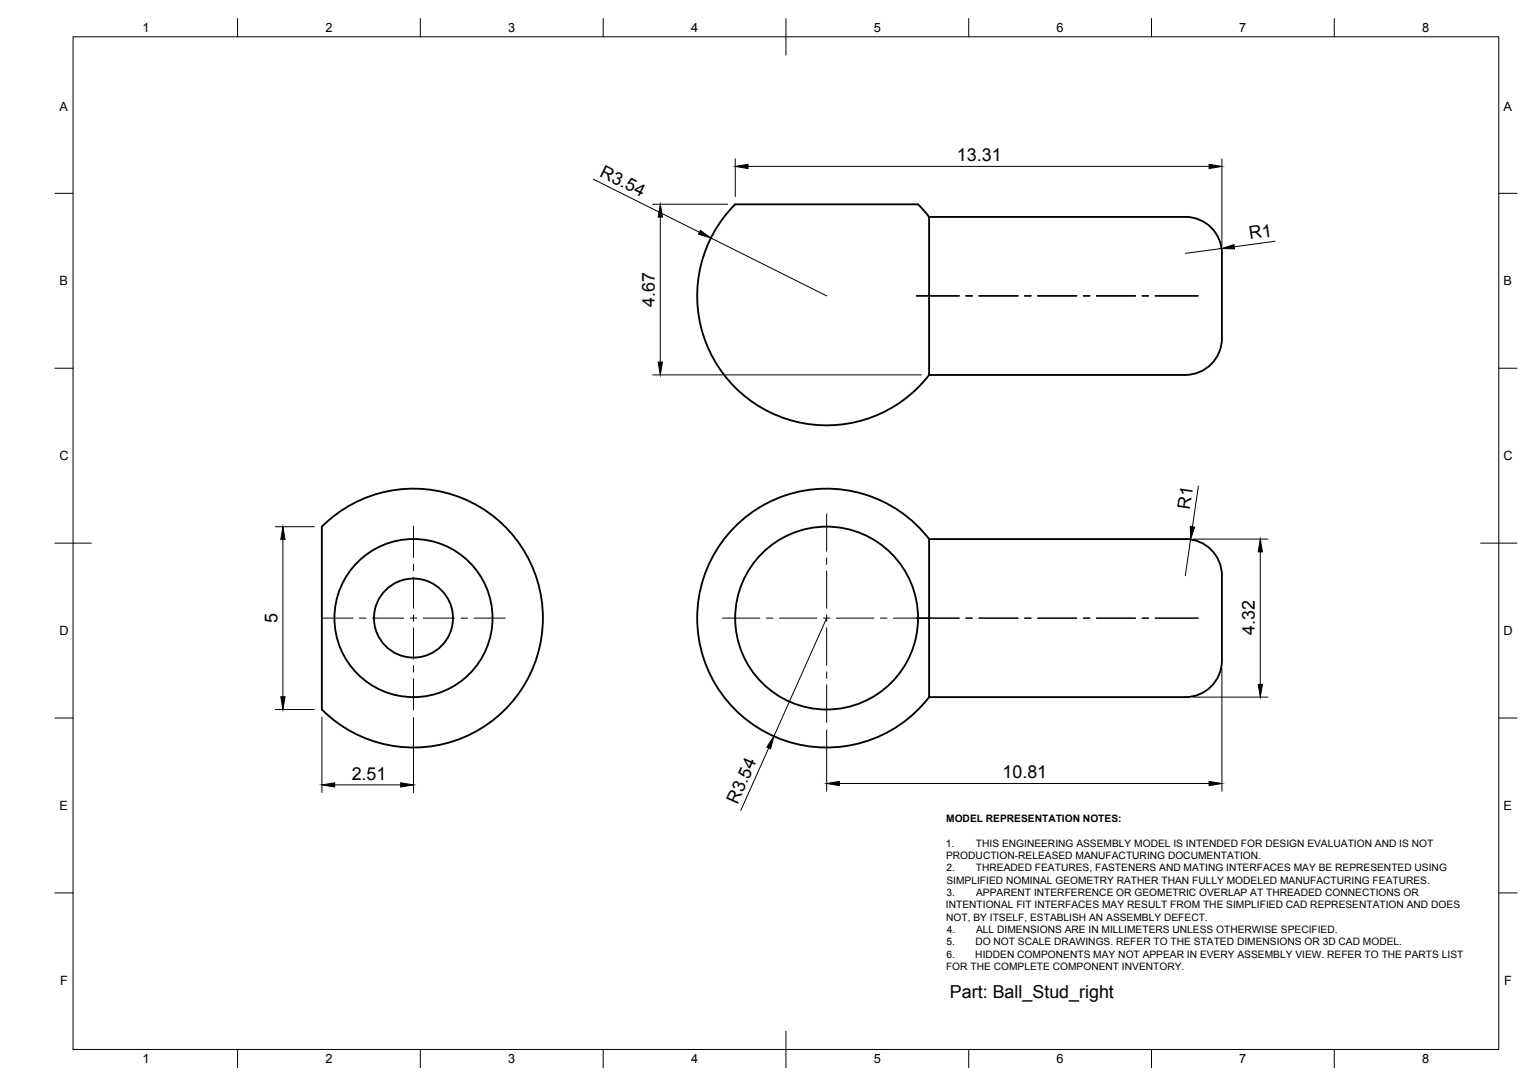
ISO-10303-21;
HEADER;
/* Generated by software containing ST-Developer
 * from STEP Tools, Inc. (www.steptools.com) 
 */

FILE_DESCRIPTION(
/* description */ (''),
/* implementation_level */ '2;1');

FILE_NAME(
/* name */ 'Ball_Stud_right.step',
/* time_stamp */ '2026-10-04T22:13:49-07:00',
/* author */ (''),
/* organization */ (''),
/* preprocessor_version */ 'ST-DEVELOPER v20.2',
/* originating_system */ 'Autodesk Translation Framework v15.15.0.0',
/* authorisation */ '');

FILE_SCHEMA (('AUTOMOTIVE_DESIGN { 1 0 10303 214 3 1 1 }'));
ENDSEC;

DATA;
#10=MECHANICAL_DESIGN_GEOMETRIC_PRESENTATION_REPRESENTATION('',(#364),#40734);
#348=SHAPE_REPRESENTATION_RELATIONSHIP('SRR','None',#40769,#356);
#356=ADVANCED_BREP_SHAPE_REPRESENTATION('',(#373),#40729);
#364=STYLED_ITEM('',(#40815),#373);
#373=MANIFOLD_SOLID_BREP('Body1',#3169);
#380=SPHERICAL_SURFACE('',#3338,3.53951905042299);
#387=FACE_BOUND('',#629,.T.);
#388=FACE_BOUND('',#634,.T.);
#394=TOROIDAL_SURFACE('',#3325,1.16126351211314,1.);
#408=PLANE('',#3324);
#409=PLANE('',#3330);
#410=PLANE('',#3337);
#459=FACE_OUTER_BOUND('',#625,.T.);
#460=FACE_OUTER_BOUND('',#626,.T.);
#461=FACE_OUTER_BOUND('',#627,.T.);
#462=FACE_OUTER_BOUND('',#628,.T.);
#463=FACE_OUTER_BOUND('',#630,.T.);
#464=FACE_OUTER_BOUND('',#631,.T.);
#465=FACE_OUTER_BOUND('',#632,.T.);
#466=FACE_OUTER_BOUND('',#633,.T.);
#625=EDGE_LOOP('',(#2088,#2089,#2090,#2091));
#626=EDGE_LOOP('',(#2092));
#627=EDGE_LOOP('',(#2093,#2094,#2095,#2096,#2097));
#628=EDGE_LOOP('',(#2098));
#629=EDGE_LOOP('',(#2099));
#630=EDGE_LOOP('',(#2100,#2101,#2102,#2103,#2104,#2105));
#631=EDGE_LOOP('',(#2106,#2107,#2108,#2109));
#632=EDGE_LOOP('',(#2110));
#633=EDGE_LOOP('',(#2111,#2112,#2113,#2114));
#634=EDGE_LOOP('',(#2115));
#786=LINE('',#6439,#928);
#787=LINE('',#6453,#929);
#788=LINE('',#6461,#930);
#928=VECTOR('',#3629,1.08063175605657);
#929=VECTOR('',#3648,2.16126351211314);
#930=VECTOR('',#3657,2.5);
#1063=CIRCLE('',#3322,1.08063175605657);
#1064=CIRCLE('',#3323,1.08063175605657);
#1065=CIRCLE('',#3326,1.16126351211314);
#1066=CIRCLE('',#3327,1.);
#1067=CIRCLE('',#3328,2.16126351211314);
#1068=CIRCLE('',#3329,2.16126351211314);
#1069=CIRCLE('',#3332,2.16126351211314);
#1070=CIRCLE('',#3333,2.16126351211314);
#1071=CIRCLE('',#3335,2.5);
#1072=CIRCLE('',#3336,2.5);
#1073=CIRCLE('',#3339,3.53951905042299);
#1149=VERTEX_POINT('',#6436);
#1150=VERTEX_POINT('',#6438);
#1151=VERTEX_POINT('',#6443);
#1152=VERTEX_POINT('',#6445);
#1153=VERTEX_POINT('',#6447);
#1154=VERTEX_POINT('',#6452);
#1155=VERTEX_POINT('',#6454);
#1156=VERTEX_POINT('',#6458);
#1157=VERTEX_POINT('',#6460);
#1158=VERTEX_POINT('',#6465);
#1520=EDGE_CURVE('',#1149,#1149,#1063,.T.);
#1521=EDGE_CURVE('',#1149,#1150,#786,.T.);
#1522=EDGE_CURVE('',#1150,#1150,#1064,.T.);
#1523=EDGE_CURVE('',#1151,#1151,#1065,.T.);
#1524=EDGE_CURVE('',#1151,#1152,#1066,.T.);
#1525=EDGE_CURVE('',#1152,#1153,#1067,.T.);
#1526=EDGE_CURVE('',#1153,#1152,#1068,.T.);
#1527=EDGE_CURVE('',#1153,#1154,#787,.T.);
#1528=EDGE_CURVE('',#1154,#1155,#1069,.T.);
#1529=EDGE_CURVE('',#1155,#1154,#1070,.T.);
#1530=EDGE_CURVE('',#1156,#1156,#1071,.T.);
#1531=EDGE_CURVE('',#1156,#1157,#788,.T.);
#1532=EDGE_CURVE('',#1157,#1157,#1072,.T.);
#1533=EDGE_CURVE('',#1155,#1158,#1073,.T.);
#2088=ORIENTED_EDGE('',*,*,#1520,.F.);
#2089=ORIENTED_EDGE('',*,*,#1521,.T.);
#2090=ORIENTED_EDGE('',*,*,#1522,.T.);
#2091=ORIENTED_EDGE('',*,*,#1521,.F.);
#2092=ORIENTED_EDGE('',*,*,#1522,.F.);
#2093=ORIENTED_EDGE('',*,*,#1523,.T.);
#2094=ORIENTED_EDGE('',*,*,#1524,.T.);
#2095=ORIENTED_EDGE('',*,*,#1525,.T.);
#2096=ORIENTED_EDGE('',*,*,#1526,.T.);
#2097=ORIENTED_EDGE('',*,*,#1524,.F.);
#2098=ORIENTED_EDGE('',*,*,#1523,.F.);
#2099=ORIENTED_EDGE('',*,*,#1520,.T.);
#2100=ORIENTED_EDGE('',*,*,#1526,.F.);
#2101=ORIENTED_EDGE('',*,*,#1527,.T.);
#2102=ORIENTED_EDGE('',*,*,#1528,.T.);
#2103=ORIENTED_EDGE('',*,*,#1529,.T.);
#2104=ORIENTED_EDGE('',*,*,#1527,.F.);
#2105=ORIENTED_EDGE('',*,*,#1525,.F.);
#2106=ORIENTED_EDGE('',*,*,#1530,.T.);
#2107=ORIENTED_EDGE('',*,*,#1531,.T.);
#2108=ORIENTED_EDGE('',*,*,#1532,.F.);
#2109=ORIENTED_EDGE('',*,*,#1531,.F.);
#2110=ORIENTED_EDGE('',*,*,#1530,.F.);
#2111=ORIENTED_EDGE('',*,*,#1529,.F.);
#2112=ORIENTED_EDGE('',*,*,#1533,.T.);
#2113=ORIENTED_EDGE('',*,*,#1533,.F.);
#2114=ORIENTED_EDGE('',*,*,#1528,.F.);
#2115=ORIENTED_EDGE('',*,*,#1532,.T.);
#2905=CYLINDRICAL_SURFACE('',#3321,1.08063175605657);
#2906=CYLINDRICAL_SURFACE('',#3331,2.16126351211314);
#2907=CYLINDRICAL_SURFACE('',#3334,2.5);
#3038=ADVANCED_FACE('',(#459),#2905,.F.);
#3039=ADVANCED_FACE('',(#460),#408,.T.);
#3040=ADVANCED_FACE('',(#461),#394,.T.);
#3041=ADVANCED_FACE('',(#462,#387),#409,.T.);
#3042=ADVANCED_FACE('',(#463),#2906,.T.);
#3043=ADVANCED_FACE('',(#464),#2907,.F.);
#3044=ADVANCED_FACE('',(#465),#410,.F.);
#3045=ADVANCED_FACE('',(#466,#388),#380,.T.);
#3169=CLOSED_SHELL('',(#3038,#3039,#3040,#3041,#3042,#3043,#3044,#3045));
#3320=AXIS2_PLACEMENT_3D('',#6434,#3623,#3624);
#3321=AXIS2_PLACEMENT_3D('',#6435,#3625,#3626);
#3322=AXIS2_PLACEMENT_3D('',#6437,#3627,#3628);
#3323=AXIS2_PLACEMENT_3D('',#6440,#3630,#3631);
#3324=AXIS2_PLACEMENT_3D('',#6441,#3632,#3633);
#3325=AXIS2_PLACEMENT_3D('',#6442,#3634,#3635);
#3326=AXIS2_PLACEMENT_3D('',#6444,#3636,#3637);
#3327=AXIS2_PLACEMENT_3D('',#6446,#3638,#3639);
#3328=AXIS2_PLACEMENT_3D('',#6448,#3640,#3641);
#3329=AXIS2_PLACEMENT_3D('',#6449,#3642,#3643);
#3330=AXIS2_PLACEMENT_3D('',#6450,#3644,#3645);
#3331=AXIS2_PLACEMENT_3D('',#6451,#3646,#3647);
#3332=AXIS2_PLACEMENT_3D('',#6455,#3649,#3650);
#3333=AXIS2_PLACEMENT_3D('',#6456,#3651,#3652);
#3334=AXIS2_PLACEMENT_3D('',#6457,#3653,#3654);
#3335=AXIS2_PLACEMENT_3D('',#6459,#3655,#3656);
#3336=AXIS2_PLACEMENT_3D('',#6462,#3658,#3659);
#3337=AXIS2_PLACEMENT_3D('',#6463,#3660,#3661);
#3338=AXIS2_PLACEMENT_3D('',#6464,#3662,#3663);
#3339=AXIS2_PLACEMENT_3D('',#6466,#3664,#3665);
#3623=DIRECTION('axis',(0.,0.,1.));
#3624=DIRECTION('refdir',(1.,0.,0.));
#3625=DIRECTION('center_axis',(1.,0.,0.));
#3626=DIRECTION('ref_axis',(0.,-1.,0.));
#3627=DIRECTION('center_axis',(1.,0.,1.22464679914735E-16));
#3628=DIRECTION('ref_axis',(0.,-1.,0.));
#3629=DIRECTION('',(1.,0.,0.));
#3630=DIRECTION('center_axis',(1.,0.,0.));
#3631=DIRECTION('ref_axis',(0.,-1.,0.));
#3632=DIRECTION('center_axis',(-1.,0.,0.));
#3633=DIRECTION('ref_axis',(0.,-1.,0.));
#3634=DIRECTION('center_axis',(-1.,0.,-1.22464679914735E-16));
#3635=DIRECTION('ref_axis',(0.,0.,1.));
#3636=DIRECTION('center_axis',(1.,0.,1.22464679914735E-16));
#3637=DIRECTION('ref_axis',(-1.22464679914735E-16,2.13056796687593E-46,
1.));
#3638=DIRECTION('center_axis',(-1.49975978266185E-32,-1.,1.22464679914735E-16));
#3639=DIRECTION('ref_axis',(0.,-1.22464679914735E-16,-1.));
#3640=DIRECTION('center_axis',(-1.,0.,-1.22464679914735E-16));
#3641=DIRECTION('ref_axis',(-1.22464679914735E-16,2.13056796687593E-46,
1.));
#3642=DIRECTION('center_axis',(-1.,0.,-1.22464679914735E-16));
#3643=DIRECTION('ref_axis',(-1.22464679914735E-16,2.13056796687593E-46,
1.));
#3644=DIRECTION('center_axis',(-1.,0.,-1.22464679914735E-16));
#3645=DIRECTION('ref_axis',(1.22464679914735E-16,-1.22464679914735E-16,
-1.));
#3646=DIRECTION('center_axis',(-1.,0.,-1.22464679914735E-16));
#3647=DIRECTION('ref_axis',(1.22464679914735E-16,-1.22464679914735E-16,
-1.));
#3648=DIRECTION('',(1.,0.,1.22464679914735E-16));
#3649=DIRECTION('center_axis',(-1.,0.,-1.22464679914735E-16));
#3650=DIRECTION('ref_axis',(1.22464679914735E-16,-1.22464679914735E-16,
-1.));
#3651=DIRECTION('center_axis',(-1.,0.,-1.22464679914735E-16));
#3652=DIRECTION('ref_axis',(1.22464679914735E-16,-1.22464679914735E-16,
-1.));
#3653=DIRECTION('center_axis',(1.22464679914735E-16,-1.22464679914735E-16,
-1.));
#3654=DIRECTION('ref_axis',(-1.,1.258548236767E-48,-1.22464679914735E-16));
#3655=DIRECTION('center_axis',(-1.22464679914735E-16,1.22464679914735E-16,
1.));
#3656=DIRECTION('ref_axis',(-1.,1.258548236767E-48,-1.22464679914735E-16));
#3657=DIRECTION('',(1.22464679914735E-16,-1.22464679914735E-16,-1.));
#3658=DIRECTION('center_axis',(-1.22464679914735E-16,1.22464679914735E-16,
1.));
#3659=DIRECTION('ref_axis',(-1.,1.258548236767E-48,-1.22464679914735E-16));
#3660=DIRECTION('center_axis',(-1.22464679914735E-16,1.22464679914735E-16,
1.));
#3661=DIRECTION('ref_axis',(-1.,1.258548236767E-48,-1.22464679914735E-16));
#3662=DIRECTION('center_axis',(-1.,1.22464679914735E-16,-1.22464679914735E-16));
#3663=DIRECTION('ref_axis',(0.,1.,-1.22464679914735E-16));
#3664=DIRECTION('center_axis',(-1.22464679914735E-16,2.4492935982947E-16,
1.));
#3665=DIRECTION('ref_axis',(0.,-1.,2.4492935982947E-16));
#6434=CARTESIAN_POINT('',(0.,0.,0.));
#6435=CARTESIAN_POINT('Origin',(85.6487002358236,0.,-8.24265256448471E-15));
#6436=CARTESIAN_POINT('',(85.6487002358236,1.08063175605657,-8.37499178659588E-15));
#6437=CARTESIAN_POINT('Origin',(85.6487002358236,0.,-8.24265256448471E-15));
#6438=CARTESIAN_POINT('',(89.1487002358236,1.08063175605657,-8.37499178659588E-15));
#6439=CARTESIAN_POINT('',(85.6487002358236,1.08063175605657,-8.11031334237355E-15));
#6440=CARTESIAN_POINT('Origin',(89.1487002358236,0.,-8.24265256448471E-15));
#6441=CARTESIAN_POINT('Origin',(89.1487002358236,0.,-8.18789480661053E-15));
#6442=CARTESIAN_POINT('Origin',(86.6487002358236,-4.60471880688602E-46,
1.0611405339408E-14));
#6443=CARTESIAN_POINT('',(85.6487002358236,1.42213764307597E-16,-1.16126351211313));
#6444=CARTESIAN_POINT('Origin',(85.6487002358236,-4.60471880688602E-46,
1.04889406594932E-14));
#6445=CARTESIAN_POINT('',(86.6487002358236,-2.64678444222332E-16,-2.16126351211313));
#6446=CARTESIAN_POINT('Origin',(86.6487002358236,-1.42213764307597E-16,
-1.16126351211313));
#6447=CARTESIAN_POINT('',(86.6487002358236,5.29356888444664E-16,2.16126351211315));
#6448=CARTESIAN_POINT('Origin',(86.6487002358236,-4.60471880688602E-46,
1.0611405339408E-14));
#6449=CARTESIAN_POINT('Origin',(86.6487002358236,-4.60471880688602E-46,
1.0611405339408E-14));
#6450=CARTESIAN_POINT('Origin',(85.6487002358236,-2.18952885050753E-46,
1.04889406594933E-14));
#6451=CARTESIAN_POINT('Origin',(89.6530615045687,-4.60471880688602E-46,
1.09793334805331E-14));
#6452=CARTESIAN_POINT('',(93.6574227733139,5.29356888444664E-16,2.16126351211315));
#6453=CARTESIAN_POINT('',(89.6530615045687,5.29356888444664E-16,2.16126351211315));
#6454=CARTESIAN_POINT('',(93.6574227733139,-2.16126351211314,1.19990831900176E-14));
#6455=CARTESIAN_POINT('Origin',(93.6574227733139,-2.18952885050753E-46,
1.14697263015729E-14));
#6456=CARTESIAN_POINT('Origin',(93.6574227733139,-2.18952885050753E-46,
1.14697263015729E-14));
#6457=CARTESIAN_POINT('Origin',(96.460480949577,-8.32667268468867E-16,1.18130019239114E-14));
#6458=CARTESIAN_POINT('',(98.960480949577,-5.26505568682029E-16,1.21191636236982E-14));
#6459=CARTESIAN_POINT('Origin',(96.460480949577,-8.32667268468867E-16,1.18130019239114E-14));
#6460=CARTESIAN_POINT('',(98.960480949577,-8.33357072363267E-16,-2.50563267625309));
#6461=CARTESIAN_POINT('',(98.960480949577,-1.13882896825571E-15,1.21191636236982E-14));
#6462=CARTESIAN_POINT('Origin',(96.460480949577,-1.13951877215011E-15,-2.50563267625309));
#6463=CARTESIAN_POINT('Origin',(96.460480949577,-6.93889390390723E-16,1.18130019239114E-14));
#6464=CARTESIAN_POINT('Origin',(96.460480949577,-2.18952885050753E-46,1.18130019239114E-14));
#6465=CARTESIAN_POINT('',(100.,-2.1673303378108E-16,1.22464679914736E-14));
#6466=CARTESIAN_POINT('Origin',(96.460480949577,-2.18952885050753E-46,1.18130019239114E-14));
#40719=UNCERTAINTY_MEASURE_WITH_UNIT(LENGTH_MEASURE(0.01),#40735,
'DISTANCE_ACCURACY_VALUE',
'Maximum model space distance between geometric entities at asserted c
onnectivities');
#40724=UNCERTAINTY_MEASURE_WITH_UNIT(LENGTH_MEASURE(0.01),#40735,
'DISTANCE_ACCURACY_VALUE',
'Maximum model space distance between geometric entities at asserted c
onnectivities');
#40729=(
GEOMETRIC_REPRESENTATION_CONTEXT(3)
GLOBAL_UNCERTAINTY_ASSIGNED_CONTEXT((#40719))
GLOBAL_UNIT_ASSIGNED_CONTEXT((#40735,#40737,#40738))
REPRESENTATION_CONTEXT('','3D')
);
#40734=(
GEOMETRIC_REPRESENTATION_CONTEXT(3)
GLOBAL_UNCERTAINTY_ASSIGNED_CONTEXT((#40724))
GLOBAL_UNIT_ASSIGNED_CONTEXT((#40735,#40737,#40738))
REPRESENTATION_CONTEXT('','3D')
);
#40735=(
LENGTH_UNIT()
NAMED_UNIT(*)
SI_UNIT(.MILLI.,.METRE.)
);
#40737=(
NAMED_UNIT(*)
PLANE_ANGLE_UNIT()
SI_UNIT($,.RADIAN.)
);
#40738=(
NAMED_UNIT(*)
SI_UNIT($,.STERADIAN.)
SOLID_ANGLE_UNIT()
);
#40743=SHAPE_DEFINITION_REPRESENTATION(#40752,#40769);
#40752=PRODUCT_DEFINITION_SHAPE('',$,#40779);
#40769=SHAPE_REPRESENTATION('',(#3320),#40729);
#40774=PRODUCT_DEFINITION_CONTEXT('part definition',#40803,'design');
#40779=PRODUCT_DEFINITION('Ball_Stud (1)','Ball_Stud_right',#40788,#40774);
#40788=PRODUCT_DEFINITION_FORMATION('',$,#40809);
#40803=APPLICATION_CONTEXT(
'Core Data for Automotive Mechanical Design Process');
#40804=PRODUCT_CONTEXT('part definition',#40803,'mechanical');
#40809=PRODUCT('Ball_Stud (1)','Ball_Stud_right',$,(#40804));
#40815=PRESENTATION_STYLE_ASSIGNMENT((#40818));
#40818=SURFACE_STYLE_USAGE(.BOTH.,#40821);
#40821=SURFACE_SIDE_STYLE('',(#40824));
#40824=SURFACE_STYLE_FILL_AREA(#40827);
#40827=FILL_AREA_STYLE('Opaque(203,203,203)',(#40830));
#40830=FILL_AREA_STYLE_COLOUR('Opaque(203,203,203)',#40833);
#40833=COLOUR_RGB('Opaque(203,203,203)', 0.09019608, 0.27058824, 0.51372549);
ENDSEC;
END-ISO-10303-21;
